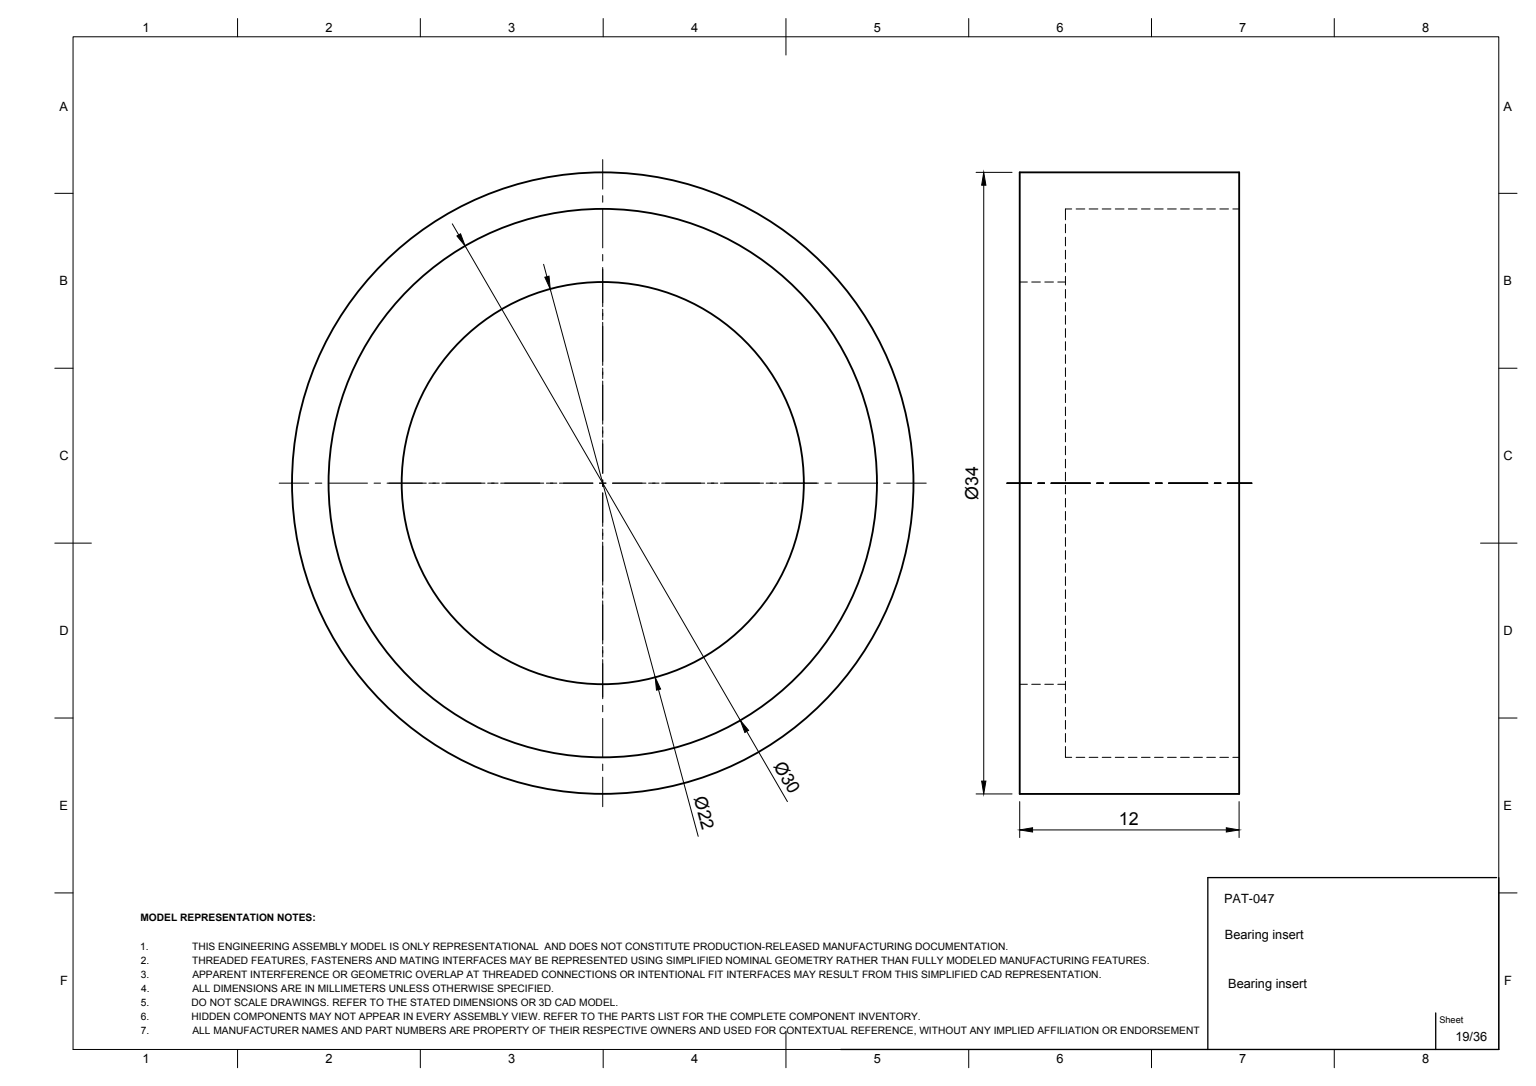
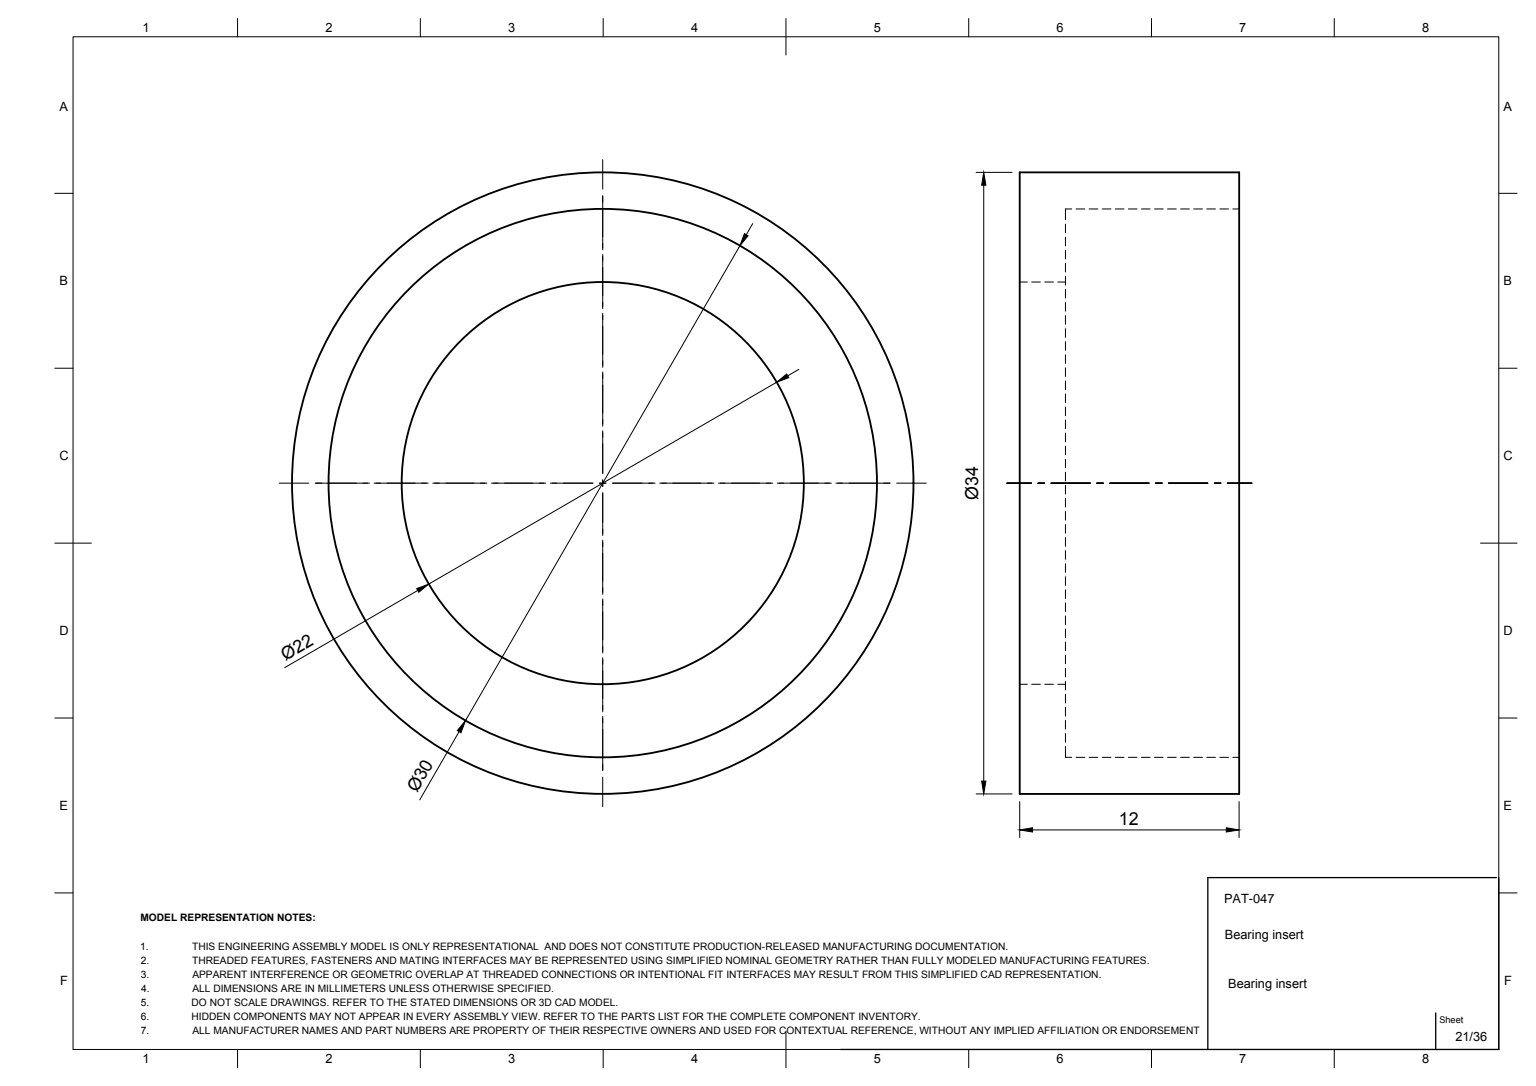
ISO-10303-21;
HEADER;
/* Generated by software containing ST-Developer
 * from STEP Tools, Inc. (www.steptools.com) 
 */

FILE_DESCRIPTION(
/* description */ ('Gravity roller conveyor section'),
/* implementation_level */ '2;1');

FILE_NAME(
/* name */ 'Bearing insert.step',
/* time_stamp */ '2026-11-02T07:43:02-08:00',
/* author */ (''),
/* organization */ (''),
/* preprocessor_version */ 'ST-DEVELOPER v20.2',
/* originating_system */ 'Autodesk Translation Framework v15.17.0.0',
/* authorisation */ '');

FILE_SCHEMA (('AUTOMOTIVE_DESIGN { 1 0 10303 214 3 1 1 }'));
ENDSEC;

DATA;
#10=MECHANICAL_DESIGN_GEOMETRIC_PRESENTATION_REPRESENTATION('',(#544),#13821);
#476=SHAPE_REPRESENTATION_RELATIONSHIP('SRR','None',#14014,#510);
#510=ADVANCED_BREP_SHAPE_REPRESENTATION('',(#584),#13801);
#544=STYLED_ITEM('',(#14191),#584);
#584=MANIFOLD_SOLID_BREP('Body1',#7644);
#652=FACE_BOUND('',#1720,.T.);
#653=FACE_BOUND('',#1724,.T.);
#654=FACE_BOUND('',#1726,.T.);
#915=PLANE('',#8379);
#916=PLANE('',#8386);
#917=PLANE('',#8387);
#1256=FACE_OUTER_BOUND('',#1718,.T.);
#1257=FACE_OUTER_BOUND('',#1719,.T.);
#1258=FACE_OUTER_BOUND('',#1721,.T.);
#1259=FACE_OUTER_BOUND('',#1722,.T.);
#1260=FACE_OUTER_BOUND('',#1723,.T.);
#1261=FACE_OUTER_BOUND('',#1725,.T.);
#1718=EDGE_LOOP('',(#6474,#6475,#6476,#6477));
#1719=EDGE_LOOP('',(#6478));
#1720=EDGE_LOOP('',(#6479));
#1721=EDGE_LOOP('',(#6480,#6481,#6482,#6483));
#1722=EDGE_LOOP('',(#6484,#6485,#6486,#6487));
#1723=EDGE_LOOP('',(#6488));
#1724=EDGE_LOOP('',(#6489));
#1725=EDGE_LOOP('',(#6490));
#1726=EDGE_LOOP('',(#6491));
#2504=LINE('',#12573,#3222);
#2505=LINE('',#12580,#3223);
#2506=LINE('',#12586,#3224);
#3222=VECTOR('',#10043,1.1);
#3223=VECTOR('',#10052,1.5);
#3224=VECTOR('',#10059,1.7);
#3434=CIRCLE('',#8377,1.1);
#3435=CIRCLE('',#8378,1.1);
#3436=CIRCLE('',#8380,1.5);
#3437=CIRCLE('',#8382,1.5);
#3438=CIRCLE('',#8384,1.7);
#3439=CIRCLE('',#8385,1.7);
#4012=VERTEX_POINT('',#12570);
#4013=VERTEX_POINT('',#12572);
#4014=VERTEX_POINT('',#12576);
#4015=VERTEX_POINT('',#12579);
#4016=VERTEX_POINT('',#12583);
#4017=VERTEX_POINT('',#12585);
#4874=EDGE_CURVE('',#4012,#4012,#3434,.T.);
#4875=EDGE_CURVE('',#4012,#4013,#2504,.T.);
#4876=EDGE_CURVE('',#4013,#4013,#3435,.T.);
#4877=EDGE_CURVE('',#4014,#4014,#3436,.T.);
#4878=EDGE_CURVE('',#4014,#4015,#2505,.T.);
#4879=EDGE_CURVE('',#4015,#4015,#3437,.T.);
#4880=EDGE_CURVE('',#4016,#4016,#3438,.T.);
#4881=EDGE_CURVE('',#4016,#4017,#2506,.T.);
#4882=EDGE_CURVE('',#4017,#4017,#3439,.T.);
#6474=ORIENTED_EDGE('',*,*,#4874,.F.);
#6475=ORIENTED_EDGE('',*,*,#4875,.T.);
#6476=ORIENTED_EDGE('',*,*,#4876,.T.);
#6477=ORIENTED_EDGE('',*,*,#4875,.F.);
#6478=ORIENTED_EDGE('',*,*,#4877,.F.);
#6479=ORIENTED_EDGE('',*,*,#4876,.F.);
#6480=ORIENTED_EDGE('',*,*,#4877,.T.);
#6481=ORIENTED_EDGE('',*,*,#4878,.T.);
#6482=ORIENTED_EDGE('',*,*,#4879,.T.);
#6483=ORIENTED_EDGE('',*,*,#4878,.F.);
#6484=ORIENTED_EDGE('',*,*,#4880,.F.);
#6485=ORIENTED_EDGE('',*,*,#4881,.T.);
#6486=ORIENTED_EDGE('',*,*,#4882,.T.);
#6487=ORIENTED_EDGE('',*,*,#4881,.F.);
#6488=ORIENTED_EDGE('',*,*,#4880,.T.);
#6489=ORIENTED_EDGE('',*,*,#4874,.T.);
#6490=ORIENTED_EDGE('',*,*,#4882,.F.);
#6491=ORIENTED_EDGE('',*,*,#4879,.F.);
#7158=CYLINDRICAL_SURFACE('',#8376,1.1);
#7159=CYLINDRICAL_SURFACE('',#8381,1.5);
#7160=CYLINDRICAL_SURFACE('',#8383,1.7);
#7457=ADVANCED_FACE('',(#1256),#7158,.F.);
#7458=ADVANCED_FACE('',(#1257,#652),#915,.F.);
#7459=ADVANCED_FACE('',(#1258),#7159,.F.);
#7460=ADVANCED_FACE('',(#1259),#7160,.T.);
#7461=ADVANCED_FACE('',(#1260,#653),#916,.T.);
#7462=ADVANCED_FACE('',(#1261,#654),#917,.F.);
#7644=CLOSED_SHELL('',(#7457,#7458,#7459,#7460,#7461,#7462));
#8375=AXIS2_PLACEMENT_3D('',#12568,#10037,#10038);
#8376=AXIS2_PLACEMENT_3D('',#12569,#10039,#10040);
#8377=AXIS2_PLACEMENT_3D('',#12571,#10041,#10042);
#8378=AXIS2_PLACEMENT_3D('',#12574,#10044,#10045);
#8379=AXIS2_PLACEMENT_3D('',#12575,#10046,#10047);
#8380=AXIS2_PLACEMENT_3D('',#12577,#10048,#10049);
#8381=AXIS2_PLACEMENT_3D('',#12578,#10050,#10051);
#8382=AXIS2_PLACEMENT_3D('',#12581,#10053,#10054);
#8383=AXIS2_PLACEMENT_3D('',#12582,#10055,#10056);
#8384=AXIS2_PLACEMENT_3D('',#12584,#10057,#10058);
#8385=AXIS2_PLACEMENT_3D('',#12587,#10060,#10061);
#8386=AXIS2_PLACEMENT_3D('',#12588,#10062,#10063);
#8387=AXIS2_PLACEMENT_3D('',#12589,#10064,#10065);
#10037=DIRECTION('axis',(0.,0.,1.));
#10038=DIRECTION('refdir',(1.,0.,0.));
#10039=DIRECTION('center_axis',(0.,1.,0.));
#10040=DIRECTION('ref_axis',(1.,0.,0.));
#10041=DIRECTION('center_axis',(0.,-1.,0.));
#10042=DIRECTION('ref_axis',(1.,0.,0.));
#10043=DIRECTION('',(0.,-1.,0.));
#10044=DIRECTION('center_axis',(0.,-1.,0.));
#10045=DIRECTION('ref_axis',(1.,0.,0.));
#10046=DIRECTION('center_axis',(0.,1.,0.));
#10047=DIRECTION('ref_axis',(1.,0.,0.));
#10048=DIRECTION('center_axis',(0.,1.,0.));
#10049=DIRECTION('ref_axis',(1.,0.,0.));
#10050=DIRECTION('center_axis',(0.,1.,0.));
#10051=DIRECTION('ref_axis',(1.,0.,0.));
#10052=DIRECTION('',(0.,-1.,0.));
#10053=DIRECTION('center_axis',(0.,-1.,0.));
#10054=DIRECTION('ref_axis',(1.,0.,0.));
#10055=DIRECTION('center_axis',(0.,1.,0.));
#10056=DIRECTION('ref_axis',(1.,0.,0.));
#10057=DIRECTION('center_axis',(0.,1.,0.));
#10058=DIRECTION('ref_axis',(1.,0.,0.));
#10059=DIRECTION('',(0.,-1.,0.));
#10060=DIRECTION('center_axis',(0.,1.,0.));
#10061=DIRECTION('ref_axis',(1.,0.,0.));
#10062=DIRECTION('center_axis',(0.,1.,0.));
#10063=DIRECTION('ref_axis',(1.,0.,0.));
#10064=DIRECTION('center_axis',(0.,1.,0.));
#10065=DIRECTION('ref_axis',(1.,0.,0.));
#12568=CARTESIAN_POINT('',(0.,0.,0.));
#12569=CARTESIAN_POINT('Origin',(3.,0.95,8.));
#12570=CARTESIAN_POINT('',(1.9,1.2,8.));
#12571=CARTESIAN_POINT('Origin',(3.,1.2,8.));
#12572=CARTESIAN_POINT('',(1.9,0.95,8.));
#12573=CARTESIAN_POINT('',(1.9,0.95,8.));
#12574=CARTESIAN_POINT('Origin',(3.,0.95,8.));
#12575=CARTESIAN_POINT('Origin',(3.,0.95,8.));
#12576=CARTESIAN_POINT('',(1.5,0.95,8.));
#12577=CARTESIAN_POINT('Origin',(3.,0.95,8.));
#12578=CARTESIAN_POINT('Origin',(3.,0.,8.));
#12579=CARTESIAN_POINT('',(1.5,0.,8.));
#12580=CARTESIAN_POINT('',(1.5,0.,8.));
#12581=CARTESIAN_POINT('Origin',(3.,0.,8.));
#12582=CARTESIAN_POINT('Origin',(3.,0.,8.));
#12583=CARTESIAN_POINT('',(1.3,1.2,8.));
#12584=CARTESIAN_POINT('Origin',(3.,1.2,8.));
#12585=CARTESIAN_POINT('',(1.3,0.,8.));
#12586=CARTESIAN_POINT('',(1.3,0.,8.));
#12587=CARTESIAN_POINT('Origin',(3.,0.,8.));
#12588=CARTESIAN_POINT('Origin',(3.,1.2,8.));
#12589=CARTESIAN_POINT('Origin',(3.,0.,8.));
#13762=UNCERTAINTY_MEASURE_WITH_UNIT(LENGTH_MEASURE(0.001),#13822,
'DISTANCE_ACCURACY_VALUE',
'Maximum model space distance between geometric entities at asserted c
onnectivities');
#13782=UNCERTAINTY_MEASURE_WITH_UNIT(LENGTH_MEASURE(0.001),#13822,
'DISTANCE_ACCURACY_VALUE',
'Maximum model space distance between geometric entities at asserted c
onnectivities');
#13801=(
GEOMETRIC_REPRESENTATION_CONTEXT(3)
GLOBAL_UNCERTAINTY_ASSIGNED_CONTEXT((#13762))
GLOBAL_UNIT_ASSIGNED_CONTEXT((#13822,#13824,#13825))
REPRESENTATION_CONTEXT('','3D')
);
#13821=(
GEOMETRIC_REPRESENTATION_CONTEXT(3)
GLOBAL_UNCERTAINTY_ASSIGNED_CONTEXT((#13782))
GLOBAL_UNIT_ASSIGNED_CONTEXT((#13822,#13824,#13825))
REPRESENTATION_CONTEXT('','3D')
);
#13822=(
LENGTH_UNIT()
NAMED_UNIT(*)
SI_UNIT(.CENTI.,.METRE.)
);
#13824=(
NAMED_UNIT(*)
PLANE_ANGLE_UNIT()
SI_UNIT($,.RADIAN.)
);
#13825=(
NAMED_UNIT(*)
SI_UNIT($,.STERADIAN.)
SOLID_ANGLE_UNIT()
);
#13844=SHAPE_DEFINITION_REPRESENTATION(#13882,#14014);
#13882=PRODUCT_DEFINITION_SHAPE('',$,#14053);
#14014=SHAPE_REPRESENTATION('',(#8375),#13801);
#14034=PRODUCT_DEFINITION_CONTEXT('part definition',#14150,'design');
#14053=PRODUCT_DEFINITION('Bearing insert','Bearing insert',#14091,#14034);
#14091=PRODUCT_DEFINITION_FORMATION('',$,#14170);
#14150=APPLICATION_CONTEXT(
'Core Data for Automotive Mechanical Design Process');
#14151=PRODUCT_CONTEXT('part definition',#14150,'mechanical');
#14170=PRODUCT('Bearing insert','Bearing insert','Bearing insert',(#14151));
#14191=PRESENTATION_STYLE_ASSIGNMENT((#14196));
#14196=SURFACE_STYLE_USAGE(.BOTH.,#14201);
#14201=SURFACE_SIDE_STYLE('',(#14206));
#14206=SURFACE_STYLE_FILL_AREA(#14211);
#14211=FILL_AREA_STYLE('CAD Library Painted - Steel gray',(#14216));
#14216=FILL_AREA_STYLE_COLOUR('CAD Library Painted - Steel gray',#14221);
#14221=COLOUR_RGB('CAD Library Painted - Steel gray',0.592156862745098,
0.631372549019608,0.67843137254902);
ENDSEC;
END-ISO-10303-21;
